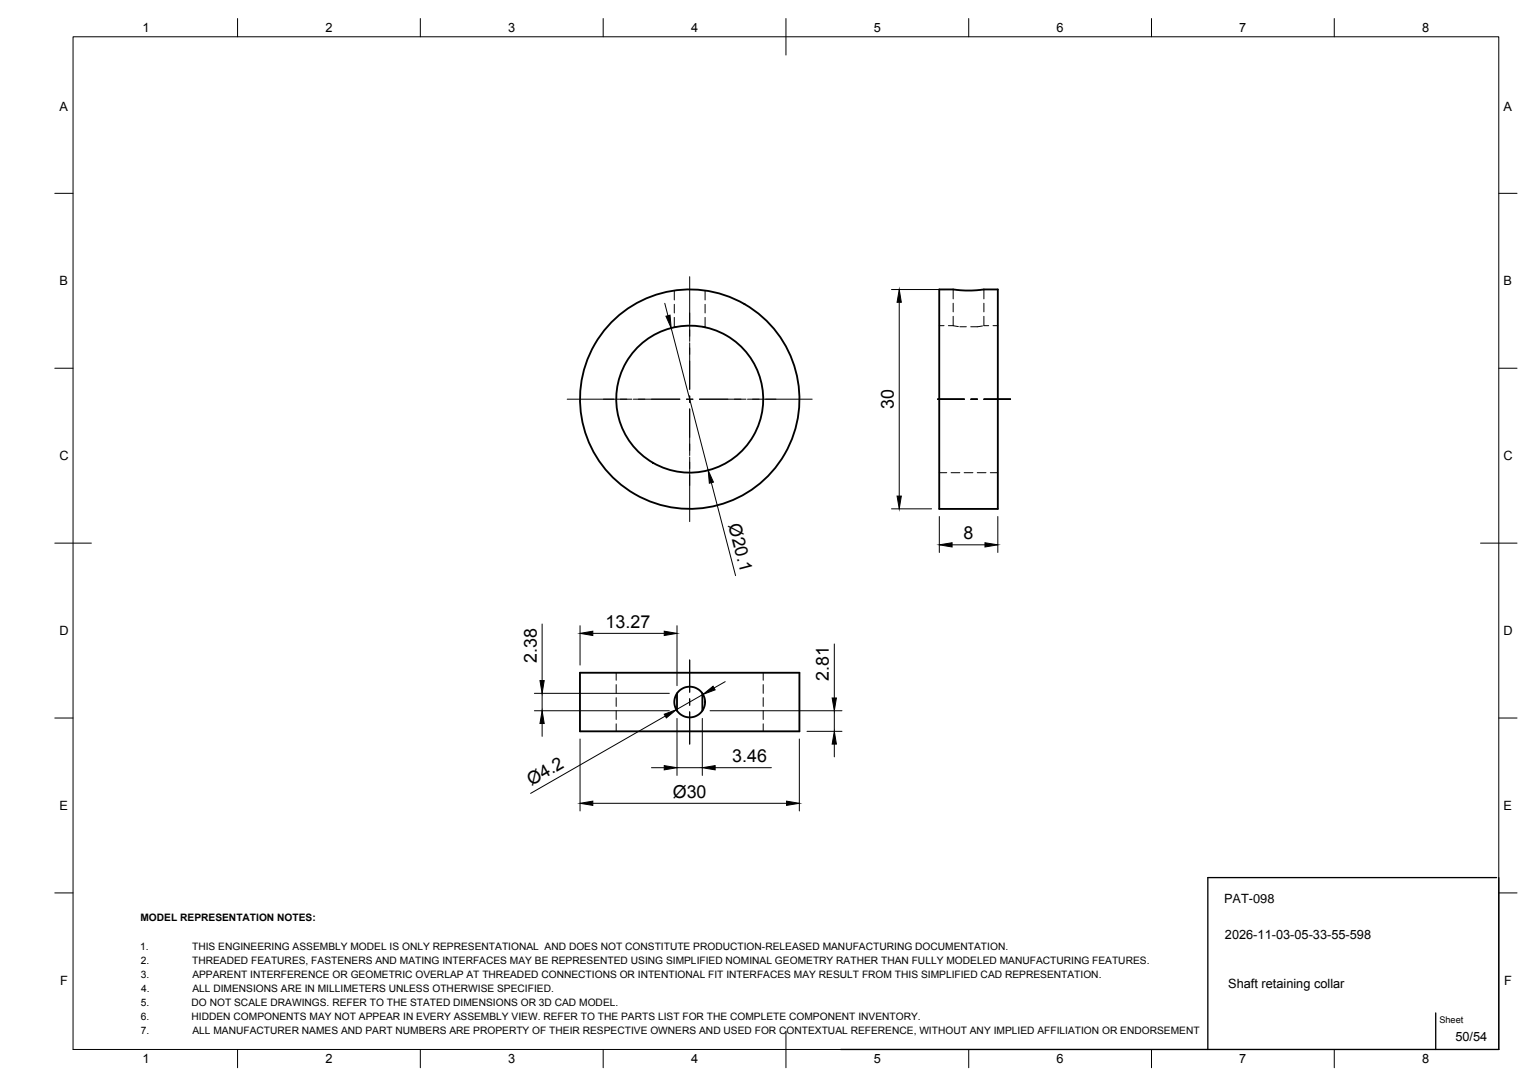
ISO-10303-21;
HEADER;
/* Generated by software containing ST-Developer
 * from STEP Tools, Inc. (www.steptools.com) 
 */

FILE_DESCRIPTION(
/* description */ ('Spring compression tester'),
/* implementation_level */ '2;1');

FILE_NAME(
/* name */ 'Shaft retaining collar.step',
/* time_stamp */ '2026-10-28T03:24:11-07:00',
/* author */ (''),
/* organization */ (''),
/* preprocessor_version */ 'ST-DEVELOPER v20.2',
/* originating_system */ 'Autodesk Translation Framework v15.17.0.0',
/* authorisation */ '');

FILE_SCHEMA (('AUTOMOTIVE_DESIGN { 1 0 10303 214 3 1 1 }'));
ENDSEC;

DATA;
#10=MECHANICAL_DESIGN_GEOMETRIC_PRESENTATION_REPRESENTATION('',(#1171),#43521);
#887=B_SPLINE_CURVE_WITH_KNOTS('',3,(#42941,#42942,#42943,#42944,#42945,
#42946,#42947,#42948),.UNSPECIFIED.,.F.,.F.,(4,2,2,4),(0.756005737987019,
0.793568827564653,0.872922520054208,0.952276212543762),.UNSPECIFIED.);
#888=B_SPLINE_CURVE_WITH_KNOTS('',3,(#42951,#42952,#42953,#42954,#42955,
#42956,#42957,#42958,#42959,#42960,#42961,#42962,#42963,#42964),
 .UNSPECIFIED.,.F.,.F.,(4,2,2,2,2,2,4),(0.121154929624509,0.158718019202145,
0.238071711691699,0.317425404181254,0.396779096670809,0.476132789160363,
0.513695878738001),.UNSPECIFIED.);
#889=B_SPLINE_CURVE_WITH_KNOTS('',3,(#42965,#42966,#42967,#42968,#42969,
#42970,#42971,#42972),.UNSPECIFIED.,.F.,.F.,(4,2,2,4),(0.952276212543762,
1.03162990503332,1.11098359752287,1.14854668710052),.UNSPECIFIED.);
#890=B_SPLINE_CURVE_WITH_KNOTS('',3,(#42976,#42977,#42978,#42979,#42980,
#42981,#42982,#42983,#42984,#42985),.UNSPECIFIED.,.F.,.F.,(4,2,2,2,4),(0.,
0.0792165807733642,0.158433161546728,0.237648697074572,0.316864232602417),
 .UNSPECIFIED.);
#891=B_SPLINE_CURVE_WITH_KNOTS('',3,(#42986,#42987,#42988,#42989,#42990,
#42991,#42992,#42993,#42994,#42995,#42996,#42997,#42998,#42999,#43000,#43001,
#43002,#43003,#43004,#43005,#43006,#43007,#43008,#43009,#43010,#43011),
 .UNSPECIFIED.,.F.,.F.,(4,2,2,2,2,2,2,2,2,2,2,2,4),(0.316864232602417,0.396079768130261,
0.475295303658105,0.554511884431469,0.633728465204833,0.712945045978197,
0.792161626751562,0.871377162279406,0.95059269780725,1.02980823333509,1.10902376886294,
1.1882403496363,1.26745693040967),.UNSPECIFIED.);
#1036=SHAPE_REPRESENTATION_RELATIONSHIP('SRR','None',#43853,#1096);
#1096=ADVANCED_BREP_SHAPE_REPRESENTATION('',(#1240),#43513);
#1171=STYLED_ITEM('',(#44202),#1240);
#1240=MANIFOLD_SOLID_BREP('Body1',#18614);
#1571=FACE_BOUND('',#4521,.T.);
#1572=FACE_BOUND('',#4523,.T.);
#1573=FACE_BOUND('',#4525,.T.);
#1574=FACE_BOUND('',#4527,.T.);
#2122=PLANE('',#21064);
#2123=PLANE('',#21068);
#2124=PLANE('',#21075);
#2125=PLANE('',#21076);
#3146=FACE_OUTER_BOUND('',#4517,.T.);
#3147=FACE_OUTER_BOUND('',#4518,.T.);
#3148=FACE_OUTER_BOUND('',#4519,.T.);
#3149=FACE_OUTER_BOUND('',#4520,.T.);
#3150=FACE_OUTER_BOUND('',#4522,.T.);
#3151=FACE_OUTER_BOUND('',#4524,.T.);
#3152=FACE_OUTER_BOUND('',#4526,.T.);
#4517=EDGE_LOOP('',(#16807,#16808));
#4518=EDGE_LOOP('',(#16809,#16810,#16811,#16812,#16813,#16814,#16815,#16816,
#16817));
#4519=EDGE_LOOP('',(#16818,#16819));
#4520=EDGE_LOOP('',(#16820,#16821,#16822,#16823));
#4521=EDGE_LOOP('',(#16824,#16825,#16826,#16827,#16828));
#4522=EDGE_LOOP('',(#16829,#16830,#16831,#16832));
#4523=EDGE_LOOP('',(#16833,#16834));
#4524=EDGE_LOOP('',(#16835));
#4525=EDGE_LOOP('',(#16836));
#4526=EDGE_LOOP('',(#16837));
#4527=EDGE_LOOP('',(#16838));
#5939=LINE('',#42936,#7371);
#5940=LINE('',#42974,#7372);
#5941=LINE('',#43013,#7373);
#5942=LINE('',#43018,#7374);
#5943=LINE('',#43024,#7375);
#7371=VECTOR('',#26091,1.);
#7372=VECTOR('',#26098,0.210000000000001);
#7373=VECTOR('',#26101,1.);
#7374=VECTOR('',#26106,1.005);
#7375=VECTOR('',#26113,1.5);
#8096=CIRCLE('',#21065,0.210000000000001);
#8097=CIRCLE('',#21067,0.210000000000001);
#8098=CIRCLE('',#21070,1.005);
#8099=CIRCLE('',#21071,1.005);
#8100=CIRCLE('',#21073,1.5);
#8101=CIRCLE('',#21074,1.5);
#9675=VERTEX_POINT('',#42934);
#9676=VERTEX_POINT('',#42935);
#9677=VERTEX_POINT('',#42939);
#9678=VERTEX_POINT('',#42940);
#9679=VERTEX_POINT('',#42949);
#9680=VERTEX_POINT('',#42973);
#9681=VERTEX_POINT('',#42975);
#9682=VERTEX_POINT('',#43015);
#9683=VERTEX_POINT('',#43017);
#9684=VERTEX_POINT('',#43021);
#9685=VERTEX_POINT('',#43023);
#12068=EDGE_CURVE('',#9675,#9676,#5939,.T.);
#12069=EDGE_CURVE('',#9675,#9676,#8096,.T.);
#12070=EDGE_CURVE('',#9677,#9678,#887,.T.);
#12071=EDGE_CURVE('',#9679,#9677,#8097,.T.);
#12072=EDGE_CURVE('',#9676,#9679,#888,.T.);
#12073=EDGE_CURVE('',#9678,#9675,#889,.T.);
#12074=EDGE_CURVE('',#9678,#9680,#5940,.T.);
#12075=EDGE_CURVE('',#9681,#9680,#890,.T.);
#12076=EDGE_CURVE('',#9680,#9681,#891,.T.);
#12077=EDGE_CURVE('',#9679,#9677,#5941,.T.);
#12078=EDGE_CURVE('',#9682,#9682,#8098,.T.);
#12079=EDGE_CURVE('',#9682,#9683,#5942,.T.);
#12080=EDGE_CURVE('',#9683,#9683,#8099,.T.);
#12081=EDGE_CURVE('',#9684,#9684,#8100,.T.);
#12082=EDGE_CURVE('',#9684,#9685,#5943,.T.);
#12083=EDGE_CURVE('',#9685,#9685,#8101,.T.);
#16807=ORIENTED_EDGE('',*,*,#12068,.F.);
#16808=ORIENTED_EDGE('',*,*,#12069,.T.);
#16809=ORIENTED_EDGE('',*,*,#12070,.F.);
#16810=ORIENTED_EDGE('',*,*,#12071,.F.);
#16811=ORIENTED_EDGE('',*,*,#12072,.F.);
#16812=ORIENTED_EDGE('',*,*,#12069,.F.);
#16813=ORIENTED_EDGE('',*,*,#12073,.F.);
#16814=ORIENTED_EDGE('',*,*,#12074,.T.);
#16815=ORIENTED_EDGE('',*,*,#12075,.F.);
#16816=ORIENTED_EDGE('',*,*,#12076,.F.);
#16817=ORIENTED_EDGE('',*,*,#12074,.F.);
#16818=ORIENTED_EDGE('',*,*,#12077,.F.);
#16819=ORIENTED_EDGE('',*,*,#12071,.T.);
#16820=ORIENTED_EDGE('',*,*,#12078,.F.);
#16821=ORIENTED_EDGE('',*,*,#12079,.T.);
#16822=ORIENTED_EDGE('',*,*,#12080,.T.);
#16823=ORIENTED_EDGE('',*,*,#12079,.F.);
#16824=ORIENTED_EDGE('',*,*,#12072,.T.);
#16825=ORIENTED_EDGE('',*,*,#12077,.T.);
#16826=ORIENTED_EDGE('',*,*,#12070,.T.);
#16827=ORIENTED_EDGE('',*,*,#12073,.T.);
#16828=ORIENTED_EDGE('',*,*,#12068,.T.);
#16829=ORIENTED_EDGE('',*,*,#12081,.F.);
#16830=ORIENTED_EDGE('',*,*,#12082,.T.);
#16831=ORIENTED_EDGE('',*,*,#12083,.T.);
#16832=ORIENTED_EDGE('',*,*,#12082,.F.);
#16833=ORIENTED_EDGE('',*,*,#12075,.T.);
#16834=ORIENTED_EDGE('',*,*,#12076,.T.);
#16835=ORIENTED_EDGE('',*,*,#12081,.T.);
#16836=ORIENTED_EDGE('',*,*,#12078,.T.);
#16837=ORIENTED_EDGE('',*,*,#12083,.F.);
#16838=ORIENTED_EDGE('',*,*,#12080,.F.);
#17477=CYLINDRICAL_SURFACE('',#21066,0.210000000000001);
#17478=CYLINDRICAL_SURFACE('',#21069,1.005);
#17479=CYLINDRICAL_SURFACE('',#21072,1.5);
#18470=ADVANCED_FACE('',(#3146),#2122,.T.);
#18471=ADVANCED_FACE('',(#3147),#17477,.F.);
#18472=ADVANCED_FACE('',(#3148),#2123,.T.);
#18473=ADVANCED_FACE('',(#3149,#1571),#17478,.F.);
#18474=ADVANCED_FACE('',(#3150,#1572),#17479,.T.);
#18475=ADVANCED_FACE('',(#3151,#1573),#2124,.T.);
#18476=ADVANCED_FACE('',(#3152,#1574),#2125,.F.);
#18614=CLOSED_SHELL('',(#18470,#18471,#18472,#18473,#18474,#18475,#18476));
#21063=AXIS2_PLACEMENT_3D('',#42932,#26087,#26088);
#21064=AXIS2_PLACEMENT_3D('',#42933,#26089,#26090);
#21065=AXIS2_PLACEMENT_3D('',#42937,#26092,#26093);
#21066=AXIS2_PLACEMENT_3D('',#42938,#26094,#26095);
#21067=AXIS2_PLACEMENT_3D('',#42950,#26096,#26097);
#21068=AXIS2_PLACEMENT_3D('',#43012,#26099,#26100);
#21069=AXIS2_PLACEMENT_3D('',#43014,#26102,#26103);
#21070=AXIS2_PLACEMENT_3D('',#43016,#26104,#26105);
#21071=AXIS2_PLACEMENT_3D('',#43019,#26107,#26108);
#21072=AXIS2_PLACEMENT_3D('',#43020,#26109,#26110);
#21073=AXIS2_PLACEMENT_3D('',#43022,#26111,#26112);
#21074=AXIS2_PLACEMENT_3D('',#43025,#26114,#26115);
#21075=AXIS2_PLACEMENT_3D('',#43026,#26116,#26117);
#21076=AXIS2_PLACEMENT_3D('',#43027,#26118,#26119);
#26087=DIRECTION('axis',(0.,0.,1.));
#26088=DIRECTION('refdir',(1.,0.,0.));
#26089=DIRECTION('center_axis',(0.,1.,0.));
#26090=DIRECTION('ref_axis',(1.,0.,0.));
#26091=DIRECTION('',(1.,0.,0.));
#26092=DIRECTION('center_axis',(0.,1.,0.));
#26093=DIRECTION('ref_axis',(1.,0.,0.));
#26094=DIRECTION('center_axis',(0.,1.,0.));
#26095=DIRECTION('ref_axis',(1.,0.,0.));
#26096=DIRECTION('center_axis',(0.,1.,0.));
#26097=DIRECTION('ref_axis',(1.,0.,0.));
#26098=DIRECTION('',(0.,1.,0.));
#26099=DIRECTION('center_axis',(0.,1.,0.));
#26100=DIRECTION('ref_axis',(1.,0.,0.));
#26101=DIRECTION('',(-1.,0.,0.));
#26102=DIRECTION('center_axis',(1.,0.,0.));
#26103=DIRECTION('ref_axis',(0.,0.,-1.));
#26104=DIRECTION('center_axis',(-1.,0.,0.));
#26105=DIRECTION('ref_axis',(0.,0.,-1.));
#26106=DIRECTION('',(-1.,0.,0.));
#26107=DIRECTION('center_axis',(-1.,0.,0.));
#26108=DIRECTION('ref_axis',(0.,0.,-1.));
#26109=DIRECTION('center_axis',(1.,0.,0.));
#26110=DIRECTION('ref_axis',(0.,0.,-1.));
#26111=DIRECTION('center_axis',(1.,0.,0.));
#26112=DIRECTION('ref_axis',(0.,0.,-1.));
#26113=DIRECTION('',(-1.,0.,0.));
#26114=DIRECTION('center_axis',(1.,0.,0.));
#26115=DIRECTION('ref_axis',(0.,0.,-1.));
#26116=DIRECTION('center_axis',(1.,0.,0.));
#26117=DIRECTION('ref_axis',(0.,0.,-1.));
#26118=DIRECTION('center_axis',(1.,0.,0.));
#26119=DIRECTION('ref_axis',(0.,0.,-1.));
#42932=CARTESIAN_POINT('',(0.,0.,0.));
#42933=CARTESIAN_POINT('Origin',(25.8,0.99,4.));
#42934=CARTESIAN_POINT('',(25.6809411910021,0.99,4.17298843892006));
#42935=CARTESIAN_POINT('',(25.9190588089979,0.99,4.17298843892006));
#42936=CARTESIAN_POINT('',(25.4,0.99,4.17298843892006));
#42937=CARTESIAN_POINT('Origin',(25.8,0.99,4.));
#42938=CARTESIAN_POINT('Origin',(25.8,0.99,4.));
#42939=CARTESIAN_POINT('',(25.6809411910021,0.99,3.82701156107994));
#42940=CARTESIAN_POINT('',(25.59,1.005,4.));
#42941=CARTESIAN_POINT('Ctrl Pts',(25.6809411910021,0.989999999999999,3.82701156107994));
#42942=CARTESIAN_POINT('Ctrl Pts',(25.6701985776047,0.99129192197638,3.83440513468868));
#42943=CARTESIAN_POINT('Ctrl Pts',(25.6603122906273,0.992653949439047,3.84270286127439));
#42944=CARTESIAN_POINT('Ctrl Pts',(25.6329072257467,0.996748084390898,3.87010792615492));
#42945=CARTESIAN_POINT('Ctrl Pts',(25.6167579436671,0.999695893276376,3.89366983224072));
#42946=CARTESIAN_POINT('Ctrl Pts',(25.5953022060351,1.00385029472357,3.94538709536759));
#42947=CARTESIAN_POINT('Ctrl Pts',(25.59,1.005,3.97354876917015));
#42948=CARTESIAN_POINT('Ctrl Pts',(25.59,1.005,4.));
#42949=CARTESIAN_POINT('',(25.9190588089979,0.99,3.82701156107994));
#42950=CARTESIAN_POINT('Origin',(25.8,0.99,4.));
#42951=CARTESIAN_POINT('Ctrl Pts',(25.9190588089979,0.99,4.17298843892006));
#42952=CARTESIAN_POINT('Ctrl Pts',(25.9298014223953,0.991291921976381,4.16559486531132));
#42953=CARTESIAN_POINT('Ctrl Pts',(25.9396877093727,0.992653949439047,4.15729713872561));
#42954=CARTESIAN_POINT('Ctrl Pts',(25.9670927742533,0.996748084390898,4.12989207384508));
#42955=CARTESIAN_POINT('Ctrl Pts',(25.9832420563329,0.999695893276376,4.10633016775929));
#42956=CARTESIAN_POINT('Ctrl Pts',(26.0046977939649,1.00385029472357,4.05461290463241));
#42957=CARTESIAN_POINT('Ctrl Pts',(26.01,1.005,4.02645123082985));
#42958=CARTESIAN_POINT('Ctrl Pts',(26.01,1.005,3.97354876917015));
#42959=CARTESIAN_POINT('Ctrl Pts',(26.0046977939649,1.00385029472357,3.94538709536759));
#42960=CARTESIAN_POINT('Ctrl Pts',(25.9832420563329,0.999695893276376,3.89366983224072));
#42961=CARTESIAN_POINT('Ctrl Pts',(25.9670927742533,0.996748084390898,3.87010792615492));
#42962=CARTESIAN_POINT('Ctrl Pts',(25.9396877093727,0.992653949439047,3.84270286127439));
#42963=CARTESIAN_POINT('Ctrl Pts',(25.9298014223953,0.991291921976381,3.83440513468868));
#42964=CARTESIAN_POINT('Ctrl Pts',(25.9190588089979,0.99,3.82701156107994));
#42965=CARTESIAN_POINT('Ctrl Pts',(25.59,1.005,4.));
#42966=CARTESIAN_POINT('Ctrl Pts',(25.59,1.005,4.02645123082985));
#42967=CARTESIAN_POINT('Ctrl Pts',(25.5953022060351,1.00385029472357,4.05461290463241));
#42968=CARTESIAN_POINT('Ctrl Pts',(25.6167579436671,0.999695893276376,4.10633016775929));
#42969=CARTESIAN_POINT('Ctrl Pts',(25.6329072257467,0.996748084390898,4.12989207384508));
#42970=CARTESIAN_POINT('Ctrl Pts',(25.6603122906273,0.992653949439047,4.15729713872561));
#42971=CARTESIAN_POINT('Ctrl Pts',(25.6701985776047,0.991291921976381,4.16559486531132));
#42972=CARTESIAN_POINT('Ctrl Pts',(25.6809411910021,0.99,4.17298843892006));
#42973=CARTESIAN_POINT('',(25.59,1.5,4.));
#42974=CARTESIAN_POINT('',(25.59,0.99,4.));
#42975=CARTESIAN_POINT('',(25.8,1.48522725533839,4.21));
#42976=CARTESIAN_POINT('Ctrl Pts',(25.8,1.48522725533839,4.21));
#42977=CARTESIAN_POINT('Ctrl Pts',(25.7735944730755,1.48522725533839,4.21));
#42978=CARTESIAN_POINT('Ctrl Pts',(25.7454529259093,1.48600415954412,4.2047157372696));
#42979=CARTESIAN_POINT('Ctrl Pts',(25.6937237310949,1.48880073282317,4.18327376303633));
#42980=CARTESIAN_POINT('Ctrl Pts',(25.670133075872,1.49077897157582,4.16711792397039));
#42981=CARTESIAN_POINT('Ctrl Pts',(25.632882321789,1.49448481141327,4.12986716988737));
#42982=CARTESIAN_POINT('Ctrl Pts',(25.6167262899986,1.49645455657129,4.10627640830577));
#42983=CARTESIAN_POINT('Ctrl Pts',(25.5952841751738,1.49923165515646,4.0545468514059));
#42984=CARTESIAN_POINT('Ctrl Pts',(25.59,1.5,4.02640517850928));
#42985=CARTESIAN_POINT('Ctrl Pts',(25.59,1.5,4.));
#42986=CARTESIAN_POINT('Ctrl Pts',(25.59,1.5,4.));
#42987=CARTESIAN_POINT('Ctrl Pts',(25.59,1.5,3.97359482149072));
#42988=CARTESIAN_POINT('Ctrl Pts',(25.5952841751738,1.49923165515646,3.9454531485941));
#42989=CARTESIAN_POINT('Ctrl Pts',(25.6167262899986,1.49645455657129,3.89372359169423));
#42990=CARTESIAN_POINT('Ctrl Pts',(25.632882321789,1.49448481141327,3.87013283011263));
#42991=CARTESIAN_POINT('Ctrl Pts',(25.670133075872,1.49077897157582,3.83288207602961));
#42992=CARTESIAN_POINT('Ctrl Pts',(25.6937237310949,1.48880073282317,3.81672623696366));
#42993=CARTESIAN_POINT('Ctrl Pts',(25.7454529259093,1.48600415954412,3.7952842627304));
#42994=CARTESIAN_POINT('Ctrl Pts',(25.7735944730755,1.48522725533839,3.79));
#42995=CARTESIAN_POINT('Ctrl Pts',(25.8264055269245,1.48522725533839,3.79));
#42996=CARTESIAN_POINT('Ctrl Pts',(25.8545470740907,1.48600415954412,3.7952842627304));
#42997=CARTESIAN_POINT('Ctrl Pts',(25.9062762689051,1.48880073282317,3.81672623696367));
#42998=CARTESIAN_POINT('Ctrl Pts',(25.929866924128,1.49077897157582,3.83288207602961));
#42999=CARTESIAN_POINT('Ctrl Pts',(25.967117678211,1.49448481141327,3.87013283011263));
#43000=CARTESIAN_POINT('Ctrl Pts',(25.9832737100014,1.49645455657129,3.89372359169423));
#43001=CARTESIAN_POINT('Ctrl Pts',(26.0047158248262,1.49923165515646,3.9454531485941));
#43002=CARTESIAN_POINT('Ctrl Pts',(26.01,1.5,3.97359482149072));
#43003=CARTESIAN_POINT('Ctrl Pts',(26.01,1.5,4.02640517850928));
#43004=CARTESIAN_POINT('Ctrl Pts',(26.0047158248262,1.49923165515646,4.0545468514059));
#43005=CARTESIAN_POINT('Ctrl Pts',(25.9832737100014,1.49645455657129,4.10627640830577));
#43006=CARTESIAN_POINT('Ctrl Pts',(25.967117678211,1.49448481141327,4.12986716988737));
#43007=CARTESIAN_POINT('Ctrl Pts',(25.929866924128,1.49077897157582,4.16711792397039));
#43008=CARTESIAN_POINT('Ctrl Pts',(25.9062762689051,1.48880073282317,4.18327376303633));
#43009=CARTESIAN_POINT('Ctrl Pts',(25.8545470740907,1.48600415954412,4.20471573726959));
#43010=CARTESIAN_POINT('Ctrl Pts',(25.8264055269245,1.48522725533839,4.21));
#43011=CARTESIAN_POINT('Ctrl Pts',(25.8,1.48522725533839,4.21));
#43012=CARTESIAN_POINT('Origin',(25.8,0.99,4.));
#43013=CARTESIAN_POINT('',(25.4,0.99,3.82701156107994));
#43014=CARTESIAN_POINT('Origin',(25.4,0.,4.));
#43015=CARTESIAN_POINT('',(26.2,-1.23077003314309E-16,5.005));
#43016=CARTESIAN_POINT('Origin',(26.2,0.,4.));
#43017=CARTESIAN_POINT('',(25.4,-1.23077003314309E-16,5.005));
#43018=CARTESIAN_POINT('',(25.4,-1.23077003314309E-16,5.005));
#43019=CARTESIAN_POINT('Origin',(25.4,0.,4.));
#43020=CARTESIAN_POINT('Origin',(25.4,0.,4.));
#43021=CARTESIAN_POINT('',(26.2,-1.83697019872103E-16,5.5));
#43022=CARTESIAN_POINT('Origin',(26.2,0.,4.));
#43023=CARTESIAN_POINT('',(25.4,-1.83697019872103E-16,5.5));
#43024=CARTESIAN_POINT('',(25.4,-1.83697019872103E-16,5.5));
#43025=CARTESIAN_POINT('Origin',(25.4,0.,4.));
#43026=CARTESIAN_POINT('Origin',(26.2,0.,4.));
#43027=CARTESIAN_POINT('Origin',(25.4,0.,4.));
#43445=UNCERTAINTY_MEASURE_WITH_UNIT(LENGTH_MEASURE(0.001),#43522,
'DISTANCE_ACCURACY_VALUE',
'Maximum model space distance between geometric entities at asserted c
onnectivities');
#43453=UNCERTAINTY_MEASURE_WITH_UNIT(LENGTH_MEASURE(0.001),#43522,
'DISTANCE_ACCURACY_VALUE',
'Maximum model space distance between geometric entities at asserted c
onnectivities');
#43513=(
GEOMETRIC_REPRESENTATION_CONTEXT(3)
GLOBAL_UNCERTAINTY_ASSIGNED_CONTEXT((#43445))
GLOBAL_UNIT_ASSIGNED_CONTEXT((#43522,#43524,#43525))
REPRESENTATION_CONTEXT('','3D')
);
#43521=(
GEOMETRIC_REPRESENTATION_CONTEXT(3)
GLOBAL_UNCERTAINTY_ASSIGNED_CONTEXT((#43453))
GLOBAL_UNIT_ASSIGNED_CONTEXT((#43522,#43524,#43525))
REPRESENTATION_CONTEXT('','3D')
);
#43522=(
LENGTH_UNIT()
NAMED_UNIT(*)
SI_UNIT(.CENTI.,.METRE.)
);
#43524=(
NAMED_UNIT(*)
PLANE_ANGLE_UNIT()
SI_UNIT($,.RADIAN.)
);
#43525=(
NAMED_UNIT(*)
SI_UNIT($,.STERADIAN.)
SOLID_ANGLE_UNIT()
);
#43585=SHAPE_DEFINITION_REPRESENTATION(#43772,#43853);
#43772=PRODUCT_DEFINITION_SHAPE('',$,#43921);
#43853=SHAPE_REPRESENTATION('',(#21063),#43513);
#43861=PRODUCT_DEFINITION_CONTEXT('part definition',#44064,'design');
#43921=PRODUCT_DEFINITION('Shaft retaining collar',
'Shaft retaining collar',#43988,#43861);
#43988=PRODUCT_DEFINITION_FORMATION('',$,#44125);
#44064=APPLICATION_CONTEXT(
'Core Data for Automotive Mechanical Design Process');
#44065=PRODUCT_CONTEXT('part definition',#44064,'mechanical');
#44125=PRODUCT('Shaft retaining collar','Shaft retaining collar',
'Shaft retaining collar',(#44065));
#44196=COLOUR_RGB('Grey',0.48,0.52,0.57);
#44197=FILL_AREA_STYLE_COLOUR('',#44196);
#44198=FILL_AREA_STYLE('',(#44197));
#44199=SURFACE_STYLE_FILL_AREA(#44198);
#44200=SURFACE_SIDE_STYLE('',(#44199));
#44201=SURFACE_STYLE_USAGE(.BOTH.,#44200);
#44202=PRESENTATION_STYLE_ASSIGNMENT((#44201));
ENDSEC;
END-ISO-10303-21;
